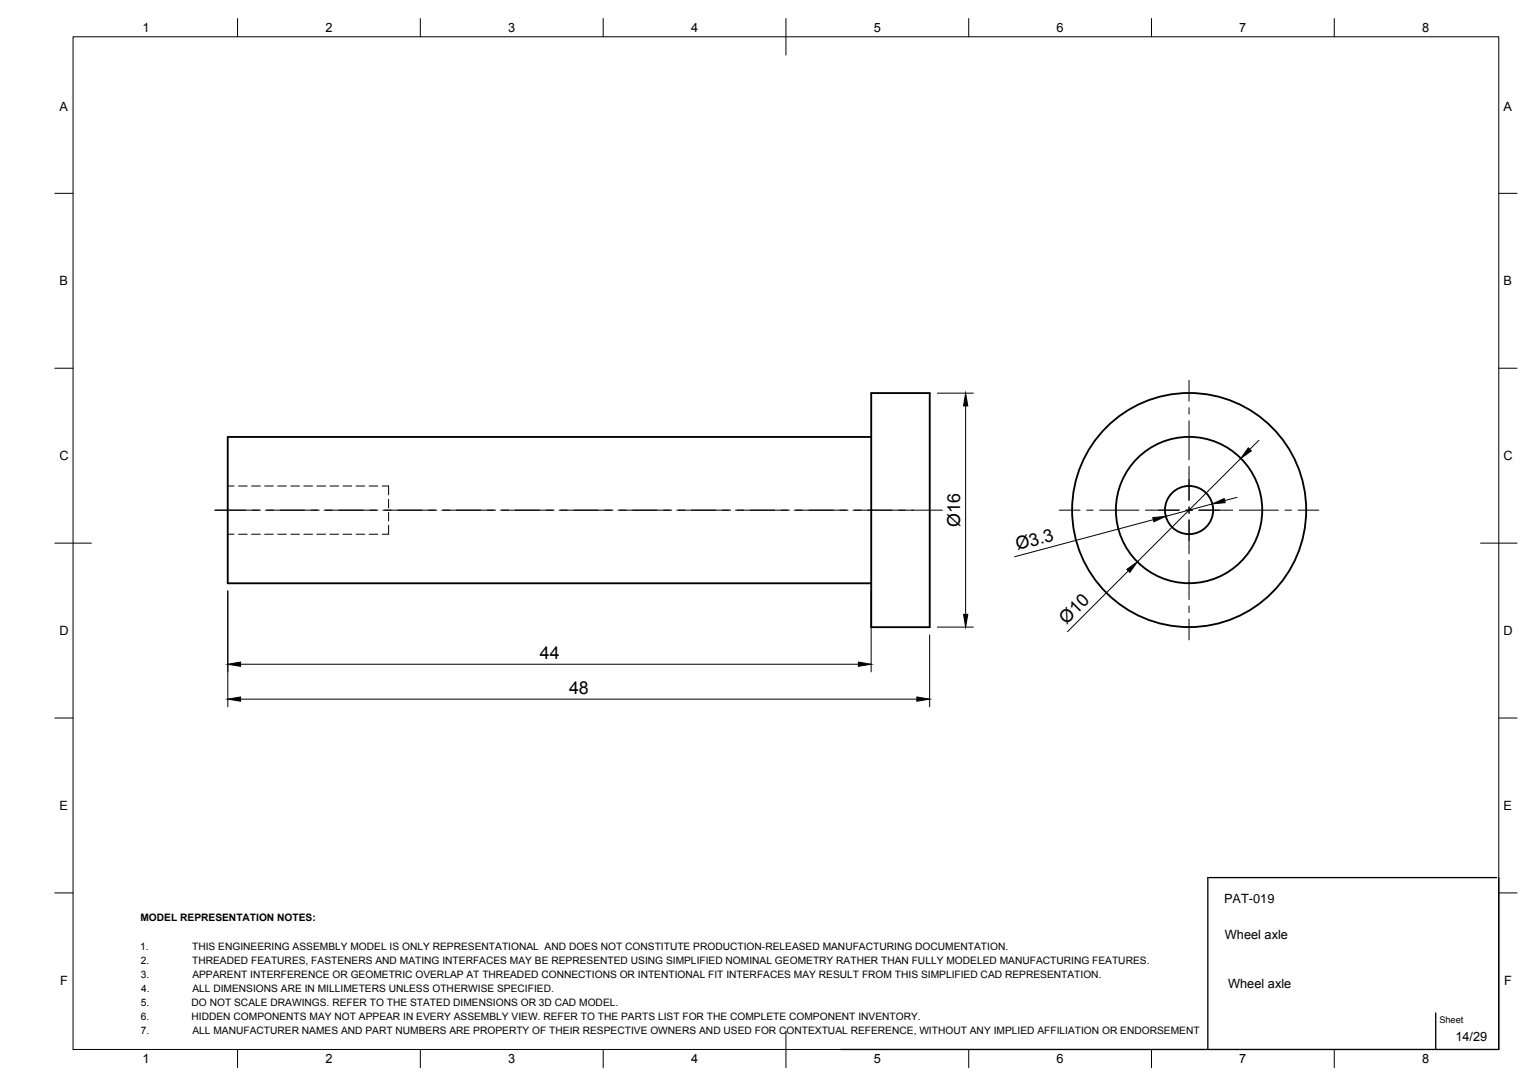
ISO-10303-21;
HEADER;
/* Generated by software containing ST-Developer
 * from STEP Tools, Inc. (www.steptools.com) 
 */

FILE_DESCRIPTION(
/* description */ ('Caster wheel assembly'),
/* implementation_level */ '2;1');

FILE_NAME(
/* name */ 'Wheel axle.step',
/* time_stamp */ '2026-10-28T03:23:56-07:00',
/* author */ (''),
/* organization */ (''),
/* preprocessor_version */ 'ST-DEVELOPER v20.2',
/* originating_system */ 'Autodesk Translation Framework v15.17.0.0',
/* authorisation */ '');

FILE_SCHEMA (('AUTOMOTIVE_DESIGN { 1 0 10303 214 3 1 1 }'));
ENDSEC;

DATA;
#10=MECHANICAL_DESIGN_GEOMETRIC_PRESENTATION_REPRESENTATION('',(#231),#5385);
#187=SHAPE_REPRESENTATION_RELATIONSHIP('SRR','None',#5483,#209);
#209=ADVANCED_BREP_SHAPE_REPRESENTATION('',(#261),#5370);
#231=STYLED_ITEM('',(#5672),#261);
#261=MANIFOLD_SOLID_BREP('Body1',#2658);
#307=FACE_BOUND('',#684,.T.);
#308=FACE_BOUND('',#689,.T.);
#375=PLANE('',#3056);
#376=PLANE('',#3057);
#377=PLANE('',#3062);
#378=PLANE('',#3065);
#487=FACE_OUTER_BOUND('',#681,.T.);
#488=FACE_OUTER_BOUND('',#682,.T.);
#489=FACE_OUTER_BOUND('',#683,.T.);
#490=FACE_OUTER_BOUND('',#685,.T.);
#491=FACE_OUTER_BOUND('',#686,.T.);
#492=FACE_OUTER_BOUND('',#687,.T.);
#493=FACE_OUTER_BOUND('',#688,.T.);
#681=EDGE_LOOP('',(#2054,#2055,#2056,#2057));
#682=EDGE_LOOP('',(#2058));
#683=EDGE_LOOP('',(#2059));
#684=EDGE_LOOP('',(#2060));
#685=EDGE_LOOP('',(#2061,#2062,#2063,#2064));
#686=EDGE_LOOP('',(#2065));
#687=EDGE_LOOP('',(#2066,#2067,#2068,#2069));
#688=EDGE_LOOP('',(#2070));
#689=EDGE_LOOP('',(#2071));
#887=LINE('',#4538,#1021);
#888=LINE('',#4548,#1022);
#889=LINE('',#4554,#1023);
#1021=VECTOR('',#3646,0.165);
#1022=VECTOR('',#3659,0.8);
#1023=VECTOR('',#3668,0.5);
#1123=CIRCLE('',#3054,0.165);
#1124=CIRCLE('',#3055,0.165);
#1125=CIRCLE('',#3058,0.8);
#1126=CIRCLE('',#3059,0.5);
#1127=CIRCLE('',#3061,0.8);
#1128=CIRCLE('',#3064,0.5);
#1326=VERTEX_POINT('',#4535);
#1327=VERTEX_POINT('',#4537);
#1328=VERTEX_POINT('',#4542);
#1329=VERTEX_POINT('',#4544);
#1330=VERTEX_POINT('',#4547);
#1331=VERTEX_POINT('',#4552);
#1595=EDGE_CURVE('',#1326,#1326,#1123,.T.);
#1596=EDGE_CURVE('',#1326,#1327,#887,.T.);
#1597=EDGE_CURVE('',#1327,#1327,#1124,.T.);
#1598=EDGE_CURVE('',#1328,#1328,#1125,.T.);
#1599=EDGE_CURVE('',#1329,#1329,#1126,.T.);
#1600=EDGE_CURVE('',#1328,#1330,#888,.T.);
#1601=EDGE_CURVE('',#1330,#1330,#1127,.T.);
#1602=EDGE_CURVE('',#1331,#1331,#1128,.T.);
#1603=EDGE_CURVE('',#1331,#1329,#889,.T.);
#2054=ORIENTED_EDGE('',*,*,#1595,.F.);
#2055=ORIENTED_EDGE('',*,*,#1596,.T.);
#2056=ORIENTED_EDGE('',*,*,#1597,.F.);
#2057=ORIENTED_EDGE('',*,*,#1596,.F.);
#2058=ORIENTED_EDGE('',*,*,#1595,.T.);
#2059=ORIENTED_EDGE('',*,*,#1598,.T.);
#2060=ORIENTED_EDGE('',*,*,#1599,.F.);
#2061=ORIENTED_EDGE('',*,*,#1598,.F.);
#2062=ORIENTED_EDGE('',*,*,#1600,.T.);
#2063=ORIENTED_EDGE('',*,*,#1601,.T.);
#2064=ORIENTED_EDGE('',*,*,#1600,.F.);
#2065=ORIENTED_EDGE('',*,*,#1601,.F.);
#2066=ORIENTED_EDGE('',*,*,#1602,.F.);
#2067=ORIENTED_EDGE('',*,*,#1603,.T.);
#2068=ORIENTED_EDGE('',*,*,#1599,.T.);
#2069=ORIENTED_EDGE('',*,*,#1603,.F.);
#2070=ORIENTED_EDGE('',*,*,#1602,.T.);
#2071=ORIENTED_EDGE('',*,*,#1597,.T.);
#2450=CYLINDRICAL_SURFACE('',#3053,0.165);
#2451=CYLINDRICAL_SURFACE('',#3060,0.8);
#2452=CYLINDRICAL_SURFACE('',#3063,0.5);
#2547=ADVANCED_FACE('',(#487),#2450,.F.);
#2548=ADVANCED_FACE('',(#488),#375,.T.);
#2549=ADVANCED_FACE('',(#489,#307),#376,.T.);
#2550=ADVANCED_FACE('',(#490),#2451,.T.);
#2551=ADVANCED_FACE('',(#491),#377,.F.);
#2552=ADVANCED_FACE('',(#492),#2452,.T.);
#2553=ADVANCED_FACE('',(#493,#308),#378,.T.);
#2658=CLOSED_SHELL('',(#2547,#2548,#2549,#2550,#2551,#2552,#2553));
#3052=AXIS2_PLACEMENT_3D('',#4533,#3640,#3641);
#3053=AXIS2_PLACEMENT_3D('',#4534,#3642,#3643);
#3054=AXIS2_PLACEMENT_3D('',#4536,#3644,#3645);
#3055=AXIS2_PLACEMENT_3D('',#4539,#3647,#3648);
#3056=AXIS2_PLACEMENT_3D('',#4540,#3649,#3650);
#3057=AXIS2_PLACEMENT_3D('',#4541,#3651,#3652);
#3058=AXIS2_PLACEMENT_3D('',#4543,#3653,#3654);
#3059=AXIS2_PLACEMENT_3D('',#4545,#3655,#3656);
#3060=AXIS2_PLACEMENT_3D('',#4546,#3657,#3658);
#3061=AXIS2_PLACEMENT_3D('',#4549,#3660,#3661);
#3062=AXIS2_PLACEMENT_3D('',#4550,#3662,#3663);
#3063=AXIS2_PLACEMENT_3D('',#4551,#3664,#3665);
#3064=AXIS2_PLACEMENT_3D('',#4553,#3666,#3667);
#3065=AXIS2_PLACEMENT_3D('',#4555,#3669,#3670);
#3640=DIRECTION('axis',(0.,0.,1.));
#3641=DIRECTION('refdir',(1.,0.,0.));
#3642=DIRECTION('center_axis',(0.,1.,0.));
#3643=DIRECTION('ref_axis',(1.,0.,0.));
#3644=DIRECTION('center_axis',(0.,1.,0.));
#3645=DIRECTION('ref_axis',(1.,0.,0.));
#3646=DIRECTION('',(0.,1.,0.));
#3647=DIRECTION('center_axis',(0.,-1.,0.));
#3648=DIRECTION('ref_axis',(1.,0.,0.));
#3649=DIRECTION('center_axis',(0.,1.,0.));
#3650=DIRECTION('ref_axis',(1.,0.,0.));
#3651=DIRECTION('center_axis',(0.,1.,0.));
#3652=DIRECTION('ref_axis',(1.,0.,0.));
#3653=DIRECTION('center_axis',(0.,1.,0.));
#3654=DIRECTION('ref_axis',(1.,0.,0.));
#3655=DIRECTION('center_axis',(0.,1.,0.));
#3656=DIRECTION('ref_axis',(1.,0.,0.));
#3657=DIRECTION('center_axis',(0.,1.,0.));
#3658=DIRECTION('ref_axis',(1.,0.,0.));
#3659=DIRECTION('',(0.,-1.,0.));
#3660=DIRECTION('center_axis',(0.,1.,0.));
#3661=DIRECTION('ref_axis',(1.,0.,0.));
#3662=DIRECTION('center_axis',(0.,1.,0.));
#3663=DIRECTION('ref_axis',(1.,0.,0.));
#3664=DIRECTION('center_axis',(0.,1.,0.));
#3665=DIRECTION('ref_axis',(1.,0.,0.));
#3666=DIRECTION('center_axis',(0.,1.,0.));
#3667=DIRECTION('ref_axis',(1.,0.,0.));
#3668=DIRECTION('',(0.,-1.,0.));
#3669=DIRECTION('center_axis',(0.,1.,0.));
#3670=DIRECTION('ref_axis',(1.,0.,0.));
#4533=CARTESIAN_POINT('',(0.,0.,0.));
#4534=CARTESIAN_POINT('Origin',(0.,1.1,4.));
#4535=CARTESIAN_POINT('',(-0.165,1.1,4.));
#4536=CARTESIAN_POINT('Origin',(0.,1.1,4.));
#4537=CARTESIAN_POINT('',(-0.165,2.2,4.));
#4538=CARTESIAN_POINT('',(-0.165,1.1,4.));
#4539=CARTESIAN_POINT('Origin',(0.,2.2,4.));
#4540=CARTESIAN_POINT('Origin',(0.,1.1,4.));
#4541=CARTESIAN_POINT('Origin',(0.,-2.2,4.));
#4542=CARTESIAN_POINT('',(-0.8,-2.2,4.));
#4543=CARTESIAN_POINT('Origin',(0.,-2.2,4.));
#4544=CARTESIAN_POINT('',(-0.5,-2.2,4.));
#4545=CARTESIAN_POINT('Origin',(0.,-2.2,4.));
#4546=CARTESIAN_POINT('Origin',(0.,-2.6,4.));
#4547=CARTESIAN_POINT('',(-0.8,-2.6,4.));
#4548=CARTESIAN_POINT('',(-0.8,-2.6,4.));
#4549=CARTESIAN_POINT('Origin',(0.,-2.6,4.));
#4550=CARTESIAN_POINT('Origin',(0.,-2.6,4.));
#4551=CARTESIAN_POINT('Origin',(0.,-2.2,4.));
#4552=CARTESIAN_POINT('',(-0.5,2.2,4.));
#4553=CARTESIAN_POINT('Origin',(0.,2.2,4.));
#4554=CARTESIAN_POINT('',(-0.5,-2.2,4.));
#4555=CARTESIAN_POINT('Origin',(0.,2.2,4.));
#5342=UNCERTAINTY_MEASURE_WITH_UNIT(LENGTH_MEASURE(0.001),#5386,
'DISTANCE_ACCURACY_VALUE',
'Maximum model space distance between geometric entities at asserted c
onnectivities');
#5357=UNCERTAINTY_MEASURE_WITH_UNIT(LENGTH_MEASURE(0.001),#5386,
'DISTANCE_ACCURACY_VALUE',
'Maximum model space distance between geometric entities at asserted c
onnectivities');
#5370=(
GEOMETRIC_REPRESENTATION_CONTEXT(3)
GLOBAL_UNCERTAINTY_ASSIGNED_CONTEXT((#5342))
GLOBAL_UNIT_ASSIGNED_CONTEXT((#5386,#5388,#5389))
REPRESENTATION_CONTEXT('','3D')
);
#5385=(
GEOMETRIC_REPRESENTATION_CONTEXT(3)
GLOBAL_UNCERTAINTY_ASSIGNED_CONTEXT((#5357))
GLOBAL_UNIT_ASSIGNED_CONTEXT((#5386,#5388,#5389))
REPRESENTATION_CONTEXT('','3D')
);
#5386=(
LENGTH_UNIT()
NAMED_UNIT(*)
SI_UNIT(.CENTI.,.METRE.)
);
#5388=(
NAMED_UNIT(*)
PLANE_ANGLE_UNIT()
SI_UNIT($,.RADIAN.)
);
#5389=(
NAMED_UNIT(*)
SI_UNIT($,.STERADIAN.)
SOLID_ANGLE_UNIT()
);
#5402=SHAPE_DEFINITION_REPRESENTATION(#5434,#5483);
#5434=PRODUCT_DEFINITION_SHAPE('',$,#5511);
#5483=SHAPE_REPRESENTATION('',(#3052),#5370);
#5498=PRODUCT_DEFINITION_CONTEXT('part definition',#5581,'design');
#5511=PRODUCT_DEFINITION('Wheel axle','Wheel axle',#5538,#5498);
#5538=PRODUCT_DEFINITION_FORMATION('',$,#5595);
#5581=APPLICATION_CONTEXT(
'Core Data for Automotive Mechanical Design Process');
#5582=PRODUCT_CONTEXT('part definition',#5581,'mechanical');
#5595=PRODUCT('Wheel axle','Wheel axle','Wheel axle',(#5582));
#5666=COLOUR_RGB('Grey',0.48,0.52,0.57);
#5667=FILL_AREA_STYLE_COLOUR('',#5666);
#5668=FILL_AREA_STYLE('',(#5667));
#5669=SURFACE_STYLE_FILL_AREA(#5668);
#5670=SURFACE_SIDE_STYLE('',(#5669));
#5671=SURFACE_STYLE_USAGE(.BOTH.,#5670);
#5672=PRESENTATION_STYLE_ASSIGNMENT((#5671));
ENDSEC;
END-ISO-10303-21;
